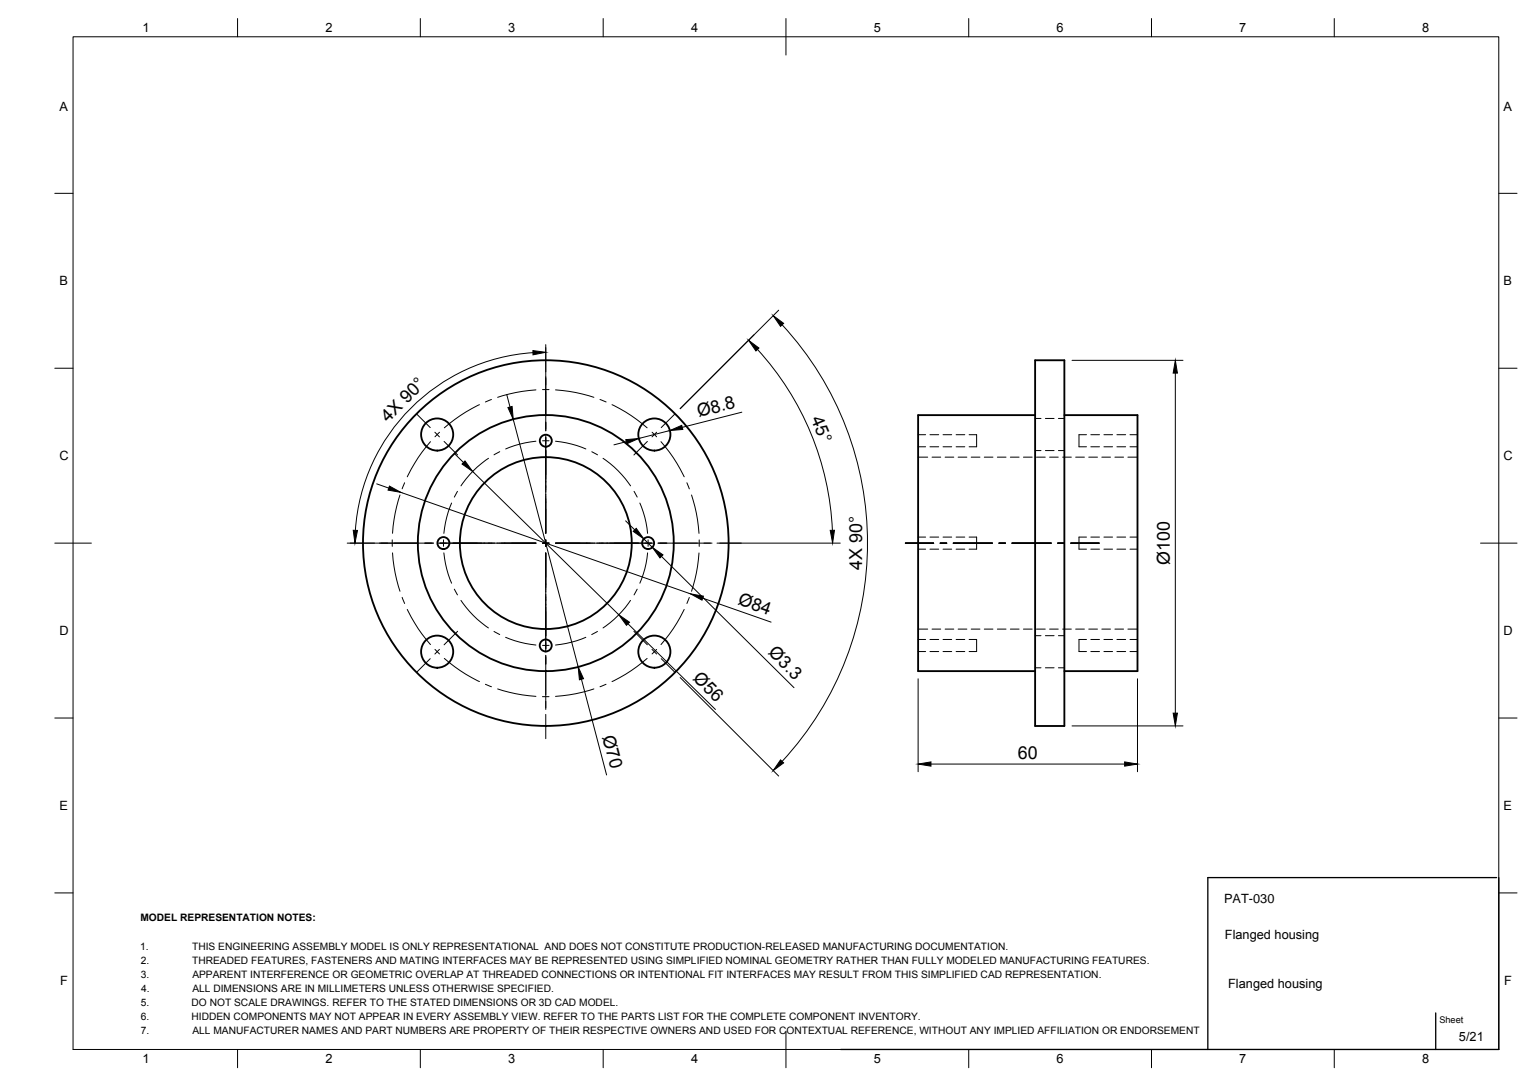
ISO-10303-21;
HEADER;
/* Generated by software containing ST-Developer
 * from STEP Tools, Inc. (www.steptools.com) 
 */

FILE_DESCRIPTION(
/* description */ ('Double-bearing flanged cartridge'),
/* implementation_level */ '2;1');

FILE_NAME(
/* name */ 'Flanged housing.step',
/* time_stamp */ '2026-10-28T03:26:40-07:00',
/* author */ (''),
/* organization */ (''),
/* preprocessor_version */ 'ST-DEVELOPER v20.2',
/* originating_system */ 'Autodesk Translation Framework v15.17.0.0',
/* authorisation */ '');

FILE_SCHEMA (('AUTOMOTIVE_DESIGN { 1 0 10303 214 3 1 1 }'));
ENDSEC;

DATA;
#10=MECHANICAL_DESIGN_GEOMETRIC_PRESENTATION_REPRESENTATION('',(#190),#5535);
#162=SHAPE_REPRESENTATION_RELATIONSHIP('SRR','None',#5603,#176);
#176=ADVANCED_BREP_SHAPE_REPRESENTATION('',(#212),#5519);
#190=STYLED_ITEM('',(#5743),#212);
#212=MANIFOLD_SOLID_BREP('Body1',#2324);
#233=FACE_BOUND('',#531,.T.);
#234=FACE_BOUND('',#532,.T.);
#235=FACE_BOUND('',#533,.T.);
#236=FACE_BOUND('',#534,.T.);
#237=FACE_BOUND('',#535,.T.);
#238=FACE_BOUND('',#537,.T.);
#239=FACE_BOUND('',#538,.T.);
#240=FACE_BOUND('',#539,.T.);
#241=FACE_BOUND('',#540,.T.);
#242=FACE_BOUND('',#541,.T.);
#243=FACE_BOUND('',#547,.T.);
#244=FACE_BOUND('',#548,.T.);
#245=FACE_BOUND('',#549,.T.);
#246=FACE_BOUND('',#550,.T.);
#247=FACE_BOUND('',#551,.T.);
#248=FACE_BOUND('',#553,.T.);
#249=FACE_BOUND('',#554,.T.);
#250=FACE_BOUND('',#555,.T.);
#251=FACE_BOUND('',#556,.T.);
#252=FACE_BOUND('',#557,.T.);
#300=PLANE('',#2520);
#301=PLANE('',#2524);
#302=PLANE('',#2528);
#303=PLANE('',#2532);
#304=PLANE('',#2536);
#305=PLANE('',#2540);
#306=PLANE('',#2544);
#307=PLANE('',#2548);
#308=PLANE('',#2549);
#309=PLANE('',#2552);
#310=PLANE('',#2563);
#311=PLANE('',#2564);
#361=FACE_OUTER_BOUND('',#510,.T.);
#362=FACE_OUTER_BOUND('',#511,.T.);
#363=FACE_OUTER_BOUND('',#512,.T.);
#364=FACE_OUTER_BOUND('',#513,.T.);
#365=FACE_OUTER_BOUND('',#514,.T.);
#366=FACE_OUTER_BOUND('',#515,.T.);
#367=FACE_OUTER_BOUND('',#516,.T.);
#368=FACE_OUTER_BOUND('',#517,.T.);
#369=FACE_OUTER_BOUND('',#518,.T.);
#370=FACE_OUTER_BOUND('',#519,.T.);
#371=FACE_OUTER_BOUND('',#520,.T.);
#372=FACE_OUTER_BOUND('',#521,.T.);
#373=FACE_OUTER_BOUND('',#522,.T.);
#374=FACE_OUTER_BOUND('',#523,.T.);
#375=FACE_OUTER_BOUND('',#524,.T.);
#376=FACE_OUTER_BOUND('',#525,.T.);
#377=FACE_OUTER_BOUND('',#526,.T.);
#378=FACE_OUTER_BOUND('',#527,.T.);
#379=FACE_OUTER_BOUND('',#528,.T.);
#380=FACE_OUTER_BOUND('',#529,.T.);
#381=FACE_OUTER_BOUND('',#530,.T.);
#382=FACE_OUTER_BOUND('',#536,.T.);
#383=FACE_OUTER_BOUND('',#542,.T.);
#384=FACE_OUTER_BOUND('',#543,.T.);
#385=FACE_OUTER_BOUND('',#544,.T.);
#386=FACE_OUTER_BOUND('',#545,.T.);
#387=FACE_OUTER_BOUND('',#546,.T.);
#388=FACE_OUTER_BOUND('',#552,.T.);
#510=EDGE_LOOP('',(#1550,#1551,#1552,#1553));
#511=EDGE_LOOP('',(#1554,#1555,#1556,#1557));
#512=EDGE_LOOP('',(#1558,#1559,#1560,#1561));
#513=EDGE_LOOP('',(#1562,#1563,#1564,#1565));
#514=EDGE_LOOP('',(#1566,#1567,#1568,#1569));
#515=EDGE_LOOP('',(#1570));
#516=EDGE_LOOP('',(#1571,#1572,#1573,#1574));
#517=EDGE_LOOP('',(#1575));
#518=EDGE_LOOP('',(#1576,#1577,#1578,#1579));
#519=EDGE_LOOP('',(#1580));
#520=EDGE_LOOP('',(#1581,#1582,#1583,#1584));
#521=EDGE_LOOP('',(#1585));
#522=EDGE_LOOP('',(#1586,#1587,#1588,#1589));
#523=EDGE_LOOP('',(#1590));
#524=EDGE_LOOP('',(#1591,#1592,#1593,#1594));
#525=EDGE_LOOP('',(#1595));
#526=EDGE_LOOP('',(#1596,#1597,#1598,#1599));
#527=EDGE_LOOP('',(#1600));
#528=EDGE_LOOP('',(#1601,#1602,#1603,#1604));
#529=EDGE_LOOP('',(#1605));
#530=EDGE_LOOP('',(#1606));
#531=EDGE_LOOP('',(#1607));
#532=EDGE_LOOP('',(#1608));
#533=EDGE_LOOP('',(#1609));
#534=EDGE_LOOP('',(#1610));
#535=EDGE_LOOP('',(#1611));
#536=EDGE_LOOP('',(#1612));
#537=EDGE_LOOP('',(#1613));
#538=EDGE_LOOP('',(#1614));
#539=EDGE_LOOP('',(#1615));
#540=EDGE_LOOP('',(#1616));
#541=EDGE_LOOP('',(#1617));
#542=EDGE_LOOP('',(#1618,#1619,#1620,#1621));
#543=EDGE_LOOP('',(#1622,#1623,#1624,#1625));
#544=EDGE_LOOP('',(#1626,#1627,#1628,#1629));
#545=EDGE_LOOP('',(#1630,#1631,#1632,#1633));
#546=EDGE_LOOP('',(#1634));
#547=EDGE_LOOP('',(#1635));
#548=EDGE_LOOP('',(#1636));
#549=EDGE_LOOP('',(#1637));
#550=EDGE_LOOP('',(#1638));
#551=EDGE_LOOP('',(#1639));
#552=EDGE_LOOP('',(#1640));
#553=EDGE_LOOP('',(#1641));
#554=EDGE_LOOP('',(#1642));
#555=EDGE_LOOP('',(#1643));
#556=EDGE_LOOP('',(#1644));
#557=EDGE_LOOP('',(#1645));
#726=LINE('',#3690,#812);
#727=LINE('',#3696,#813);
#728=LINE('',#3702,#814);
#729=LINE('',#3708,#815);
#730=LINE('',#3714,#816);
#731=LINE('',#3721,#817);
#732=LINE('',#3728,#818);
#733=LINE('',#3735,#819);
#734=LINE('',#3742,#820);
#735=LINE('',#3749,#821);
#736=LINE('',#3756,#822);
#737=LINE('',#3763,#823);
#738=LINE('',#3777,#824);
#739=LINE('',#3780,#825);
#740=LINE('',#3786,#826);
#741=LINE('',#3791,#827);
#812=VECTOR('',#2877,0.44);
#813=VECTOR('',#2884,0.44);
#814=VECTOR('',#2891,0.44);
#815=VECTOR('',#2898,0.44);
#816=VECTOR('',#2905,0.165);
#817=VECTOR('',#2914,0.165);
#818=VECTOR('',#2923,0.165);
#819=VECTOR('',#2932,0.165);
#820=VECTOR('',#2941,0.165);
#821=VECTOR('',#2950,0.165);
#822=VECTOR('',#2959,0.165);
#823=VECTOR('',#2968,0.165);
#824=VECTOR('',#2987,5.);
#825=VECTOR('',#2990,3.5);
#826=VECTOR('',#2997,2.35);
#827=VECTOR('',#3004,3.5);
#898=CIRCLE('',#2506,0.44);
#899=CIRCLE('',#2507,0.44);
#900=CIRCLE('',#2509,0.44);
#901=CIRCLE('',#2510,0.44);
#902=CIRCLE('',#2512,0.44);
#903=CIRCLE('',#2513,0.44);
#904=CIRCLE('',#2515,0.44);
#905=CIRCLE('',#2516,0.44);
#906=CIRCLE('',#2518,0.165);
#907=CIRCLE('',#2519,0.165);
#908=CIRCLE('',#2522,0.165);
#909=CIRCLE('',#2523,0.165);
#910=CIRCLE('',#2526,0.165);
#911=CIRCLE('',#2527,0.165);
#912=CIRCLE('',#2530,0.165);
#913=CIRCLE('',#2531,0.165);
#914=CIRCLE('',#2534,0.165);
#915=CIRCLE('',#2535,0.165);
#916=CIRCLE('',#2538,0.165);
#917=CIRCLE('',#2539,0.165);
#918=CIRCLE('',#2542,0.165);
#919=CIRCLE('',#2543,0.165);
#920=CIRCLE('',#2546,0.165);
#921=CIRCLE('',#2547,0.165);
#922=CIRCLE('',#2550,5.);
#923=CIRCLE('',#2551,3.5);
#924=CIRCLE('',#2553,5.);
#925=CIRCLE('',#2554,3.5);
#926=CIRCLE('',#2557,3.5);
#927=CIRCLE('',#2559,2.35);
#928=CIRCLE('',#2560,2.35);
#929=CIRCLE('',#2562,3.5);
#1072=VERTEX_POINT('',#3687);
#1073=VERTEX_POINT('',#3689);
#1074=VERTEX_POINT('',#3693);
#1075=VERTEX_POINT('',#3695);
#1076=VERTEX_POINT('',#3699);
#1077=VERTEX_POINT('',#3701);
#1078=VERTEX_POINT('',#3705);
#1079=VERTEX_POINT('',#3707);
#1080=VERTEX_POINT('',#3711);
#1081=VERTEX_POINT('',#3713);
#1082=VERTEX_POINT('',#3718);
#1083=VERTEX_POINT('',#3720);
#1084=VERTEX_POINT('',#3725);
#1085=VERTEX_POINT('',#3727);
#1086=VERTEX_POINT('',#3732);
#1087=VERTEX_POINT('',#3734);
#1088=VERTEX_POINT('',#3739);
#1089=VERTEX_POINT('',#3741);
#1090=VERTEX_POINT('',#3746);
#1091=VERTEX_POINT('',#3748);
#1092=VERTEX_POINT('',#3753);
#1093=VERTEX_POINT('',#3755);
#1094=VERTEX_POINT('',#3760);
#1095=VERTEX_POINT('',#3762);
#1096=VERTEX_POINT('',#3767);
#1097=VERTEX_POINT('',#3769);
#1098=VERTEX_POINT('',#3772);
#1099=VERTEX_POINT('',#3774);
#1100=VERTEX_POINT('',#3779);
#1101=VERTEX_POINT('',#3783);
#1102=VERTEX_POINT('',#3785);
#1103=VERTEX_POINT('',#3789);
#1268=EDGE_CURVE('',#1072,#1072,#898,.T.);
#1269=EDGE_CURVE('',#1072,#1073,#726,.T.);
#1270=EDGE_CURVE('',#1073,#1073,#899,.T.);
#1271=EDGE_CURVE('',#1074,#1074,#900,.T.);
#1272=EDGE_CURVE('',#1074,#1075,#727,.T.);
#1273=EDGE_CURVE('',#1075,#1075,#901,.T.);
#1274=EDGE_CURVE('',#1076,#1076,#902,.T.);
#1275=EDGE_CURVE('',#1076,#1077,#728,.T.);
#1276=EDGE_CURVE('',#1077,#1077,#903,.T.);
#1277=EDGE_CURVE('',#1078,#1078,#904,.T.);
#1278=EDGE_CURVE('',#1078,#1079,#729,.T.);
#1279=EDGE_CURVE('',#1079,#1079,#905,.T.);
#1280=EDGE_CURVE('',#1080,#1080,#906,.T.);
#1281=EDGE_CURVE('',#1080,#1081,#730,.T.);
#1282=EDGE_CURVE('',#1081,#1081,#907,.T.);
#1283=EDGE_CURVE('',#1082,#1082,#908,.T.);
#1284=EDGE_CURVE('',#1082,#1083,#731,.T.);
#1285=EDGE_CURVE('',#1083,#1083,#909,.T.);
#1286=EDGE_CURVE('',#1084,#1084,#910,.T.);
#1287=EDGE_CURVE('',#1084,#1085,#732,.T.);
#1288=EDGE_CURVE('',#1085,#1085,#911,.T.);
#1289=EDGE_CURVE('',#1086,#1086,#912,.T.);
#1290=EDGE_CURVE('',#1086,#1087,#733,.T.);
#1291=EDGE_CURVE('',#1087,#1087,#913,.T.);
#1292=EDGE_CURVE('',#1088,#1088,#914,.T.);
#1293=EDGE_CURVE('',#1088,#1089,#734,.T.);
#1294=EDGE_CURVE('',#1089,#1089,#915,.T.);
#1295=EDGE_CURVE('',#1090,#1090,#916,.T.);
#1296=EDGE_CURVE('',#1090,#1091,#735,.T.);
#1297=EDGE_CURVE('',#1091,#1091,#917,.T.);
#1298=EDGE_CURVE('',#1092,#1092,#918,.T.);
#1299=EDGE_CURVE('',#1092,#1093,#736,.T.);
#1300=EDGE_CURVE('',#1093,#1093,#919,.T.);
#1301=EDGE_CURVE('',#1094,#1094,#920,.T.);
#1302=EDGE_CURVE('',#1094,#1095,#737,.T.);
#1303=EDGE_CURVE('',#1095,#1095,#921,.T.);
#1304=EDGE_CURVE('',#1096,#1096,#922,.T.);
#1305=EDGE_CURVE('',#1097,#1097,#923,.T.);
#1306=EDGE_CURVE('',#1098,#1098,#924,.T.);
#1307=EDGE_CURVE('',#1099,#1099,#925,.T.);
#1308=EDGE_CURVE('',#1096,#1098,#738,.T.);
#1309=EDGE_CURVE('',#1099,#1100,#739,.T.);
#1310=EDGE_CURVE('',#1100,#1100,#926,.T.);
#1311=EDGE_CURVE('',#1101,#1101,#927,.T.);
#1312=EDGE_CURVE('',#1101,#1102,#740,.T.);
#1313=EDGE_CURVE('',#1102,#1102,#928,.T.);
#1314=EDGE_CURVE('',#1103,#1103,#929,.T.);
#1315=EDGE_CURVE('',#1103,#1097,#741,.T.);
#1550=ORIENTED_EDGE('',*,*,#1268,.F.);
#1551=ORIENTED_EDGE('',*,*,#1269,.T.);
#1552=ORIENTED_EDGE('',*,*,#1270,.F.);
#1553=ORIENTED_EDGE('',*,*,#1269,.F.);
#1554=ORIENTED_EDGE('',*,*,#1271,.F.);
#1555=ORIENTED_EDGE('',*,*,#1272,.T.);
#1556=ORIENTED_EDGE('',*,*,#1273,.F.);
#1557=ORIENTED_EDGE('',*,*,#1272,.F.);
#1558=ORIENTED_EDGE('',*,*,#1274,.F.);
#1559=ORIENTED_EDGE('',*,*,#1275,.T.);
#1560=ORIENTED_EDGE('',*,*,#1276,.F.);
#1561=ORIENTED_EDGE('',*,*,#1275,.F.);
#1562=ORIENTED_EDGE('',*,*,#1277,.F.);
#1563=ORIENTED_EDGE('',*,*,#1278,.T.);
#1564=ORIENTED_EDGE('',*,*,#1279,.F.);
#1565=ORIENTED_EDGE('',*,*,#1278,.F.);
#1566=ORIENTED_EDGE('',*,*,#1280,.F.);
#1567=ORIENTED_EDGE('',*,*,#1281,.T.);
#1568=ORIENTED_EDGE('',*,*,#1282,.F.);
#1569=ORIENTED_EDGE('',*,*,#1281,.F.);
#1570=ORIENTED_EDGE('',*,*,#1280,.T.);
#1571=ORIENTED_EDGE('',*,*,#1283,.F.);
#1572=ORIENTED_EDGE('',*,*,#1284,.T.);
#1573=ORIENTED_EDGE('',*,*,#1285,.F.);
#1574=ORIENTED_EDGE('',*,*,#1284,.F.);
#1575=ORIENTED_EDGE('',*,*,#1283,.T.);
#1576=ORIENTED_EDGE('',*,*,#1286,.F.);
#1577=ORIENTED_EDGE('',*,*,#1287,.T.);
#1578=ORIENTED_EDGE('',*,*,#1288,.F.);
#1579=ORIENTED_EDGE('',*,*,#1287,.F.);
#1580=ORIENTED_EDGE('',*,*,#1286,.T.);
#1581=ORIENTED_EDGE('',*,*,#1289,.F.);
#1582=ORIENTED_EDGE('',*,*,#1290,.T.);
#1583=ORIENTED_EDGE('',*,*,#1291,.F.);
#1584=ORIENTED_EDGE('',*,*,#1290,.F.);
#1585=ORIENTED_EDGE('',*,*,#1289,.T.);
#1586=ORIENTED_EDGE('',*,*,#1292,.F.);
#1587=ORIENTED_EDGE('',*,*,#1293,.T.);
#1588=ORIENTED_EDGE('',*,*,#1294,.T.);
#1589=ORIENTED_EDGE('',*,*,#1293,.F.);
#1590=ORIENTED_EDGE('',*,*,#1294,.F.);
#1591=ORIENTED_EDGE('',*,*,#1295,.F.);
#1592=ORIENTED_EDGE('',*,*,#1296,.T.);
#1593=ORIENTED_EDGE('',*,*,#1297,.T.);
#1594=ORIENTED_EDGE('',*,*,#1296,.F.);
#1595=ORIENTED_EDGE('',*,*,#1297,.F.);
#1596=ORIENTED_EDGE('',*,*,#1298,.F.);
#1597=ORIENTED_EDGE('',*,*,#1299,.T.);
#1598=ORIENTED_EDGE('',*,*,#1300,.T.);
#1599=ORIENTED_EDGE('',*,*,#1299,.F.);
#1600=ORIENTED_EDGE('',*,*,#1300,.F.);
#1601=ORIENTED_EDGE('',*,*,#1301,.F.);
#1602=ORIENTED_EDGE('',*,*,#1302,.T.);
#1603=ORIENTED_EDGE('',*,*,#1303,.T.);
#1604=ORIENTED_EDGE('',*,*,#1302,.F.);
#1605=ORIENTED_EDGE('',*,*,#1303,.F.);
#1606=ORIENTED_EDGE('',*,*,#1304,.T.);
#1607=ORIENTED_EDGE('',*,*,#1305,.F.);
#1608=ORIENTED_EDGE('',*,*,#1279,.T.);
#1609=ORIENTED_EDGE('',*,*,#1276,.T.);
#1610=ORIENTED_EDGE('',*,*,#1273,.T.);
#1611=ORIENTED_EDGE('',*,*,#1270,.T.);
#1612=ORIENTED_EDGE('',*,*,#1306,.F.);
#1613=ORIENTED_EDGE('',*,*,#1307,.F.);
#1614=ORIENTED_EDGE('',*,*,#1277,.T.);
#1615=ORIENTED_EDGE('',*,*,#1274,.T.);
#1616=ORIENTED_EDGE('',*,*,#1271,.T.);
#1617=ORIENTED_EDGE('',*,*,#1268,.T.);
#1618=ORIENTED_EDGE('',*,*,#1304,.F.);
#1619=ORIENTED_EDGE('',*,*,#1308,.T.);
#1620=ORIENTED_EDGE('',*,*,#1306,.T.);
#1621=ORIENTED_EDGE('',*,*,#1308,.F.);
#1622=ORIENTED_EDGE('',*,*,#1307,.T.);
#1623=ORIENTED_EDGE('',*,*,#1309,.T.);
#1624=ORIENTED_EDGE('',*,*,#1310,.T.);
#1625=ORIENTED_EDGE('',*,*,#1309,.F.);
#1626=ORIENTED_EDGE('',*,*,#1311,.F.);
#1627=ORIENTED_EDGE('',*,*,#1312,.T.);
#1628=ORIENTED_EDGE('',*,*,#1313,.T.);
#1629=ORIENTED_EDGE('',*,*,#1312,.F.);
#1630=ORIENTED_EDGE('',*,*,#1314,.F.);
#1631=ORIENTED_EDGE('',*,*,#1315,.T.);
#1632=ORIENTED_EDGE('',*,*,#1305,.T.);
#1633=ORIENTED_EDGE('',*,*,#1315,.F.);
#1634=ORIENTED_EDGE('',*,*,#1314,.T.);
#1635=ORIENTED_EDGE('',*,*,#1311,.T.);
#1636=ORIENTED_EDGE('',*,*,#1291,.T.);
#1637=ORIENTED_EDGE('',*,*,#1288,.T.);
#1638=ORIENTED_EDGE('',*,*,#1285,.T.);
#1639=ORIENTED_EDGE('',*,*,#1282,.T.);
#1640=ORIENTED_EDGE('',*,*,#1310,.F.);
#1641=ORIENTED_EDGE('',*,*,#1313,.F.);
#1642=ORIENTED_EDGE('',*,*,#1301,.T.);
#1643=ORIENTED_EDGE('',*,*,#1298,.T.);
#1644=ORIENTED_EDGE('',*,*,#1295,.T.);
#1645=ORIENTED_EDGE('',*,*,#1292,.T.);
#2114=CYLINDRICAL_SURFACE('',#2505,0.44);
#2115=CYLINDRICAL_SURFACE('',#2508,0.44);
#2116=CYLINDRICAL_SURFACE('',#2511,0.44);
#2117=CYLINDRICAL_SURFACE('',#2514,0.44);
#2118=CYLINDRICAL_SURFACE('',#2517,0.165);
#2119=CYLINDRICAL_SURFACE('',#2521,0.165);
#2120=CYLINDRICAL_SURFACE('',#2525,0.165);
#2121=CYLINDRICAL_SURFACE('',#2529,0.165);
#2122=CYLINDRICAL_SURFACE('',#2533,0.165);
#2123=CYLINDRICAL_SURFACE('',#2537,0.165);
#2124=CYLINDRICAL_SURFACE('',#2541,0.165);
#2125=CYLINDRICAL_SURFACE('',#2545,0.165);
#2126=CYLINDRICAL_SURFACE('',#2555,5.);
#2127=CYLINDRICAL_SURFACE('',#2556,3.5);
#2128=CYLINDRICAL_SURFACE('',#2558,2.35);
#2129=CYLINDRICAL_SURFACE('',#2561,3.5);
#2175=ADVANCED_FACE('',(#361),#2114,.F.);
#2176=ADVANCED_FACE('',(#362),#2115,.F.);
#2177=ADVANCED_FACE('',(#363),#2116,.F.);
#2178=ADVANCED_FACE('',(#364),#2117,.F.);
#2179=ADVANCED_FACE('',(#365),#2118,.F.);
#2180=ADVANCED_FACE('',(#366),#300,.T.);
#2181=ADVANCED_FACE('',(#367),#2119,.F.);
#2182=ADVANCED_FACE('',(#368),#301,.T.);
#2183=ADVANCED_FACE('',(#369),#2120,.F.);
#2184=ADVANCED_FACE('',(#370),#302,.T.);
#2185=ADVANCED_FACE('',(#371),#2121,.F.);
#2186=ADVANCED_FACE('',(#372),#303,.T.);
#2187=ADVANCED_FACE('',(#373),#2122,.F.);
#2188=ADVANCED_FACE('',(#374),#304,.F.);
#2189=ADVANCED_FACE('',(#375),#2123,.F.);
#2190=ADVANCED_FACE('',(#376),#305,.F.);
#2191=ADVANCED_FACE('',(#377),#2124,.F.);
#2192=ADVANCED_FACE('',(#378),#306,.F.);
#2193=ADVANCED_FACE('',(#379),#2125,.F.);
#2194=ADVANCED_FACE('',(#380),#307,.F.);
#2195=ADVANCED_FACE('',(#381,#233,#234,#235,#236,#237),#308,.T.);
#2196=ADVANCED_FACE('',(#382,#238,#239,#240,#241,#242),#309,.F.);
#2197=ADVANCED_FACE('',(#383),#2126,.T.);
#2198=ADVANCED_FACE('',(#384),#2127,.T.);
#2199=ADVANCED_FACE('',(#385),#2128,.F.);
#2200=ADVANCED_FACE('',(#386),#2129,.T.);
#2201=ADVANCED_FACE('',(#387,#243,#244,#245,#246,#247),#310,.T.);
#2202=ADVANCED_FACE('',(#388,#248,#249,#250,#251,#252),#311,.F.);
#2324=CLOSED_SHELL('',(#2175,#2176,#2177,#2178,#2179,#2180,#2181,#2182,
#2183,#2184,#2185,#2186,#2187,#2188,#2189,#2190,#2191,#2192,#2193,#2194,
#2195,#2196,#2197,#2198,#2199,#2200,#2201,#2202));
#2504=AXIS2_PLACEMENT_3D('',#3685,#2871,#2872);
#2505=AXIS2_PLACEMENT_3D('',#3686,#2873,#2874);
#2506=AXIS2_PLACEMENT_3D('',#3688,#2875,#2876);
#2507=AXIS2_PLACEMENT_3D('',#3691,#2878,#2879);
#2508=AXIS2_PLACEMENT_3D('',#3692,#2880,#2881);
#2509=AXIS2_PLACEMENT_3D('',#3694,#2882,#2883);
#2510=AXIS2_PLACEMENT_3D('',#3697,#2885,#2886);
#2511=AXIS2_PLACEMENT_3D('',#3698,#2887,#2888);
#2512=AXIS2_PLACEMENT_3D('',#3700,#2889,#2890);
#2513=AXIS2_PLACEMENT_3D('',#3703,#2892,#2893);
#2514=AXIS2_PLACEMENT_3D('',#3704,#2894,#2895);
#2515=AXIS2_PLACEMENT_3D('',#3706,#2896,#2897);
#2516=AXIS2_PLACEMENT_3D('',#3709,#2899,#2900);
#2517=AXIS2_PLACEMENT_3D('',#3710,#2901,#2902);
#2518=AXIS2_PLACEMENT_3D('',#3712,#2903,#2904);
#2519=AXIS2_PLACEMENT_3D('',#3715,#2906,#2907);
#2520=AXIS2_PLACEMENT_3D('',#3716,#2908,#2909);
#2521=AXIS2_PLACEMENT_3D('',#3717,#2910,#2911);
#2522=AXIS2_PLACEMENT_3D('',#3719,#2912,#2913);
#2523=AXIS2_PLACEMENT_3D('',#3722,#2915,#2916);
#2524=AXIS2_PLACEMENT_3D('',#3723,#2917,#2918);
#2525=AXIS2_PLACEMENT_3D('',#3724,#2919,#2920);
#2526=AXIS2_PLACEMENT_3D('',#3726,#2921,#2922);
#2527=AXIS2_PLACEMENT_3D('',#3729,#2924,#2925);
#2528=AXIS2_PLACEMENT_3D('',#3730,#2926,#2927);
#2529=AXIS2_PLACEMENT_3D('',#3731,#2928,#2929);
#2530=AXIS2_PLACEMENT_3D('',#3733,#2930,#2931);
#2531=AXIS2_PLACEMENT_3D('',#3736,#2933,#2934);
#2532=AXIS2_PLACEMENT_3D('',#3737,#2935,#2936);
#2533=AXIS2_PLACEMENT_3D('',#3738,#2937,#2938);
#2534=AXIS2_PLACEMENT_3D('',#3740,#2939,#2940);
#2535=AXIS2_PLACEMENT_3D('',#3743,#2942,#2943);
#2536=AXIS2_PLACEMENT_3D('',#3744,#2944,#2945);
#2537=AXIS2_PLACEMENT_3D('',#3745,#2946,#2947);
#2538=AXIS2_PLACEMENT_3D('',#3747,#2948,#2949);
#2539=AXIS2_PLACEMENT_3D('',#3750,#2951,#2952);
#2540=AXIS2_PLACEMENT_3D('',#3751,#2953,#2954);
#2541=AXIS2_PLACEMENT_3D('',#3752,#2955,#2956);
#2542=AXIS2_PLACEMENT_3D('',#3754,#2957,#2958);
#2543=AXIS2_PLACEMENT_3D('',#3757,#2960,#2961);
#2544=AXIS2_PLACEMENT_3D('',#3758,#2962,#2963);
#2545=AXIS2_PLACEMENT_3D('',#3759,#2964,#2965);
#2546=AXIS2_PLACEMENT_3D('',#3761,#2966,#2967);
#2547=AXIS2_PLACEMENT_3D('',#3764,#2969,#2970);
#2548=AXIS2_PLACEMENT_3D('',#3765,#2971,#2972);
#2549=AXIS2_PLACEMENT_3D('',#3766,#2973,#2974);
#2550=AXIS2_PLACEMENT_3D('',#3768,#2975,#2976);
#2551=AXIS2_PLACEMENT_3D('',#3770,#2977,#2978);
#2552=AXIS2_PLACEMENT_3D('',#3771,#2979,#2980);
#2553=AXIS2_PLACEMENT_3D('',#3773,#2981,#2982);
#2554=AXIS2_PLACEMENT_3D('',#3775,#2983,#2984);
#2555=AXIS2_PLACEMENT_3D('',#3776,#2985,#2986);
#2556=AXIS2_PLACEMENT_3D('',#3778,#2988,#2989);
#2557=AXIS2_PLACEMENT_3D('',#3781,#2991,#2992);
#2558=AXIS2_PLACEMENT_3D('',#3782,#2993,#2994);
#2559=AXIS2_PLACEMENT_3D('',#3784,#2995,#2996);
#2560=AXIS2_PLACEMENT_3D('',#3787,#2998,#2999);
#2561=AXIS2_PLACEMENT_3D('',#3788,#3000,#3001);
#2562=AXIS2_PLACEMENT_3D('',#3790,#3002,#3003);
#2563=AXIS2_PLACEMENT_3D('',#3792,#3005,#3006);
#2564=AXIS2_PLACEMENT_3D('',#3793,#3007,#3008);
#2871=DIRECTION('axis',(0.,0.,1.));
#2872=DIRECTION('refdir',(1.,0.,0.));
#2873=DIRECTION('center_axis',(0.,1.,0.));
#2874=DIRECTION('ref_axis',(1.,0.,0.));
#2875=DIRECTION('center_axis',(0.,1.,0.));
#2876=DIRECTION('ref_axis',(1.,0.,0.));
#2877=DIRECTION('',(0.,1.,0.));
#2878=DIRECTION('center_axis',(0.,-1.,0.));
#2879=DIRECTION('ref_axis',(1.,0.,0.));
#2880=DIRECTION('center_axis',(0.,1.,0.));
#2881=DIRECTION('ref_axis',(1.,0.,0.));
#2882=DIRECTION('center_axis',(0.,1.,0.));
#2883=DIRECTION('ref_axis',(1.,0.,0.));
#2884=DIRECTION('',(0.,1.,0.));
#2885=DIRECTION('center_axis',(0.,-1.,0.));
#2886=DIRECTION('ref_axis',(1.,0.,0.));
#2887=DIRECTION('center_axis',(0.,1.,0.));
#2888=DIRECTION('ref_axis',(1.,0.,0.));
#2889=DIRECTION('center_axis',(0.,1.,0.));
#2890=DIRECTION('ref_axis',(1.,0.,0.));
#2891=DIRECTION('',(0.,1.,0.));
#2892=DIRECTION('center_axis',(0.,-1.,0.));
#2893=DIRECTION('ref_axis',(1.,0.,0.));
#2894=DIRECTION('center_axis',(0.,1.,0.));
#2895=DIRECTION('ref_axis',(1.,0.,0.));
#2896=DIRECTION('center_axis',(0.,1.,0.));
#2897=DIRECTION('ref_axis',(1.,0.,0.));
#2898=DIRECTION('',(0.,1.,0.));
#2899=DIRECTION('center_axis',(0.,-1.,0.));
#2900=DIRECTION('ref_axis',(1.,0.,0.));
#2901=DIRECTION('center_axis',(0.,1.,0.));
#2902=DIRECTION('ref_axis',(1.,0.,0.));
#2903=DIRECTION('center_axis',(0.,1.,0.));
#2904=DIRECTION('ref_axis',(1.,0.,0.));
#2905=DIRECTION('',(0.,1.,0.));
#2906=DIRECTION('center_axis',(0.,-1.,0.));
#2907=DIRECTION('ref_axis',(1.,0.,0.));
#2908=DIRECTION('center_axis',(0.,1.,0.));
#2909=DIRECTION('ref_axis',(1.,0.,0.));
#2910=DIRECTION('center_axis',(0.,1.,0.));
#2911=DIRECTION('ref_axis',(1.,0.,0.));
#2912=DIRECTION('center_axis',(0.,1.,0.));
#2913=DIRECTION('ref_axis',(1.,0.,0.));
#2914=DIRECTION('',(0.,1.,0.));
#2915=DIRECTION('center_axis',(0.,-1.,0.));
#2916=DIRECTION('ref_axis',(1.,0.,0.));
#2917=DIRECTION('center_axis',(0.,1.,0.));
#2918=DIRECTION('ref_axis',(1.,0.,0.));
#2919=DIRECTION('center_axis',(0.,1.,0.));
#2920=DIRECTION('ref_axis',(1.,0.,0.));
#2921=DIRECTION('center_axis',(0.,1.,0.));
#2922=DIRECTION('ref_axis',(1.,0.,0.));
#2923=DIRECTION('',(0.,1.,0.));
#2924=DIRECTION('center_axis',(0.,-1.,0.));
#2925=DIRECTION('ref_axis',(1.,0.,0.));
#2926=DIRECTION('center_axis',(0.,1.,0.));
#2927=DIRECTION('ref_axis',(1.,0.,0.));
#2928=DIRECTION('center_axis',(0.,1.,0.));
#2929=DIRECTION('ref_axis',(1.,0.,0.));
#2930=DIRECTION('center_axis',(0.,1.,0.));
#2931=DIRECTION('ref_axis',(1.,0.,0.));
#2932=DIRECTION('',(0.,1.,0.));
#2933=DIRECTION('center_axis',(0.,-1.,0.));
#2934=DIRECTION('ref_axis',(1.,0.,0.));
#2935=DIRECTION('center_axis',(0.,1.,0.));
#2936=DIRECTION('ref_axis',(1.,0.,0.));
#2937=DIRECTION('center_axis',(0.,1.,0.));
#2938=DIRECTION('ref_axis',(1.,0.,0.));
#2939=DIRECTION('center_axis',(0.,1.,0.));
#2940=DIRECTION('ref_axis',(1.,0.,0.));
#2941=DIRECTION('',(0.,1.,0.));
#2942=DIRECTION('center_axis',(0.,1.,0.));
#2943=DIRECTION('ref_axis',(1.,0.,0.));
#2944=DIRECTION('center_axis',(0.,1.,0.));
#2945=DIRECTION('ref_axis',(1.,0.,0.));
#2946=DIRECTION('center_axis',(0.,1.,0.));
#2947=DIRECTION('ref_axis',(1.,0.,0.));
#2948=DIRECTION('center_axis',(0.,1.,0.));
#2949=DIRECTION('ref_axis',(1.,0.,0.));
#2950=DIRECTION('',(0.,1.,0.));
#2951=DIRECTION('center_axis',(0.,1.,0.));
#2952=DIRECTION('ref_axis',(1.,0.,0.));
#2953=DIRECTION('center_axis',(0.,1.,0.));
#2954=DIRECTION('ref_axis',(1.,0.,0.));
#2955=DIRECTION('center_axis',(0.,1.,0.));
#2956=DIRECTION('ref_axis',(1.,0.,0.));
#2957=DIRECTION('center_axis',(0.,1.,0.));
#2958=DIRECTION('ref_axis',(1.,0.,0.));
#2959=DIRECTION('',(0.,1.,0.));
#2960=DIRECTION('center_axis',(0.,1.,0.));
#2961=DIRECTION('ref_axis',(1.,0.,0.));
#2962=DIRECTION('center_axis',(0.,1.,0.));
#2963=DIRECTION('ref_axis',(1.,0.,0.));
#2964=DIRECTION('center_axis',(0.,1.,0.));
#2965=DIRECTION('ref_axis',(1.,0.,0.));
#2966=DIRECTION('center_axis',(0.,1.,0.));
#2967=DIRECTION('ref_axis',(1.,0.,0.));
#2968=DIRECTION('',(0.,1.,0.));
#2969=DIRECTION('center_axis',(0.,1.,0.));
#2970=DIRECTION('ref_axis',(1.,0.,0.));
#2971=DIRECTION('center_axis',(0.,1.,0.));
#2972=DIRECTION('ref_axis',(1.,0.,0.));
#2973=DIRECTION('center_axis',(0.,1.,0.));
#2974=DIRECTION('ref_axis',(1.,0.,0.));
#2975=DIRECTION('center_axis',(0.,1.,0.));
#2976=DIRECTION('ref_axis',(1.,0.,0.));
#2977=DIRECTION('center_axis',(0.,1.,0.));
#2978=DIRECTION('ref_axis',(1.,0.,0.));
#2979=DIRECTION('center_axis',(0.,1.,0.));
#2980=DIRECTION('ref_axis',(1.,0.,0.));
#2981=DIRECTION('center_axis',(0.,1.,0.));
#2982=DIRECTION('ref_axis',(1.,0.,0.));
#2983=DIRECTION('center_axis',(0.,-1.,0.));
#2984=DIRECTION('ref_axis',(1.,0.,0.));
#2985=DIRECTION('center_axis',(0.,1.,0.));
#2986=DIRECTION('ref_axis',(1.,0.,0.));
#2987=DIRECTION('',(0.,-1.,0.));
#2988=DIRECTION('center_axis',(0.,1.,0.));
#2989=DIRECTION('ref_axis',(1.,0.,0.));
#2990=DIRECTION('',(0.,-1.,0.));
#2991=DIRECTION('center_axis',(0.,1.,0.));
#2992=DIRECTION('ref_axis',(1.,0.,0.));
#2993=DIRECTION('center_axis',(0.,1.,0.));
#2994=DIRECTION('ref_axis',(1.,0.,0.));
#2995=DIRECTION('center_axis',(0.,-1.,0.));
#2996=DIRECTION('ref_axis',(1.,0.,0.));
#2997=DIRECTION('',(0.,-1.,0.));
#2998=DIRECTION('center_axis',(0.,-1.,0.));
#2999=DIRECTION('ref_axis',(1.,0.,0.));
#3000=DIRECTION('center_axis',(0.,1.,0.));
#3001=DIRECTION('ref_axis',(1.,0.,0.));
#3002=DIRECTION('center_axis',(0.,1.,0.));
#3003=DIRECTION('ref_axis',(1.,0.,0.));
#3004=DIRECTION('',(0.,-1.,0.));
#3005=DIRECTION('center_axis',(0.,1.,0.));
#3006=DIRECTION('ref_axis',(1.,0.,0.));
#3007=DIRECTION('center_axis',(0.,1.,0.));
#3008=DIRECTION('ref_axis',(1.,0.,0.));
#3685=CARTESIAN_POINT('',(0.,0.,0.));
#3686=CARTESIAN_POINT('Origin',(-2.9698484809835,1.9,1.5301515190165));
#3687=CARTESIAN_POINT('',(-3.4098484809835,2.,1.5301515190165));
#3688=CARTESIAN_POINT('Origin',(-2.9698484809835,2.,1.5301515190165));
#3689=CARTESIAN_POINT('',(-3.4098484809835,2.8,1.5301515190165));
#3690=CARTESIAN_POINT('',(-3.4098484809835,1.9,1.5301515190165));
#3691=CARTESIAN_POINT('Origin',(-2.9698484809835,2.8,1.5301515190165));
#3692=CARTESIAN_POINT('Origin',(-2.9698484809835,1.9,7.4698484809835));
#3693=CARTESIAN_POINT('',(-3.4098484809835,2.,7.4698484809835));
#3694=CARTESIAN_POINT('Origin',(-2.9698484809835,2.,7.4698484809835));
#3695=CARTESIAN_POINT('',(-3.4098484809835,2.8,7.4698484809835));
#3696=CARTESIAN_POINT('',(-3.4098484809835,1.9,7.4698484809835));
#3697=CARTESIAN_POINT('Origin',(-2.9698484809835,2.8,7.4698484809835));
#3698=CARTESIAN_POINT('Origin',(2.9698484809835,1.9,7.4698484809835));
#3699=CARTESIAN_POINT('',(2.5298484809835,2.,7.4698484809835));
#3700=CARTESIAN_POINT('Origin',(2.9698484809835,2.,7.4698484809835));
#3701=CARTESIAN_POINT('',(2.5298484809835,2.8,7.4698484809835));
#3702=CARTESIAN_POINT('',(2.5298484809835,1.9,7.4698484809835));
#3703=CARTESIAN_POINT('Origin',(2.9698484809835,2.8,7.4698484809835));
#3704=CARTESIAN_POINT('Origin',(2.9698484809835,1.9,1.5301515190165));
#3705=CARTESIAN_POINT('',(2.5298484809835,2.,1.5301515190165));
#3706=CARTESIAN_POINT('Origin',(2.9698484809835,2.,1.5301515190165));
#3707=CARTESIAN_POINT('',(2.5298484809835,2.8,1.5301515190165));
#3708=CARTESIAN_POINT('',(2.5298484809835,1.9,1.5301515190165));
#3709=CARTESIAN_POINT('Origin',(2.9698484809835,2.8,1.5301515190165));
#3710=CARTESIAN_POINT('Origin',(-2.8,4.4,4.5));
#3711=CARTESIAN_POINT('',(-2.965,4.4,4.5));
#3712=CARTESIAN_POINT('Origin',(-2.8,4.4,4.5));
#3713=CARTESIAN_POINT('',(-2.965,6.,4.5));
#3714=CARTESIAN_POINT('',(-2.965,4.4,4.5));
#3715=CARTESIAN_POINT('Origin',(-2.8,6.,4.5));
#3716=CARTESIAN_POINT('Origin',(-2.8,4.4,4.5));
#3717=CARTESIAN_POINT('Origin',(1.71450551880629E-16,4.4,7.3));
#3718=CARTESIAN_POINT('',(-0.165,4.4,7.3));
#3719=CARTESIAN_POINT('Origin',(1.71450551880629E-16,4.4,7.3));
#3720=CARTESIAN_POINT('',(-0.165,6.,7.3));
#3721=CARTESIAN_POINT('',(-0.165,4.4,7.3));
#3722=CARTESIAN_POINT('Origin',(1.71450551880629E-16,6.,7.3));
#3723=CARTESIAN_POINT('Origin',(1.66533453693773E-16,4.4,7.3));
#3724=CARTESIAN_POINT('Origin',(2.8,4.4,4.5));
#3725=CARTESIAN_POINT('',(2.635,4.4,4.5));
#3726=CARTESIAN_POINT('Origin',(2.8,4.4,4.5));
#3727=CARTESIAN_POINT('',(2.635,6.,4.5));
#3728=CARTESIAN_POINT('',(2.635,4.4,4.5));
#3729=CARTESIAN_POINT('Origin',(2.8,6.,4.5));
#3730=CARTESIAN_POINT('Origin',(2.8,4.4,4.5));
#3731=CARTESIAN_POINT('Origin',(-5.14351655641888E-16,4.4,1.7));
#3732=CARTESIAN_POINT('',(-0.165000000000001,4.4,1.7));
#3733=CARTESIAN_POINT('Origin',(-5.14351655641888E-16,4.4,1.7));
#3734=CARTESIAN_POINT('',(-0.165000000000001,6.,1.7));
#3735=CARTESIAN_POINT('',(-0.165000000000001,4.4,1.7));
#3736=CARTESIAN_POINT('Origin',(-5.14351655641888E-16,6.,1.7));
#3737=CARTESIAN_POINT('Origin',(-5.27355936696949E-16,4.4,1.7));
#3738=CARTESIAN_POINT('Origin',(-2.8,-0.1,4.5));
#3739=CARTESIAN_POINT('',(-2.965,0.,4.5));
#3740=CARTESIAN_POINT('Origin',(-2.8,0.,4.5));
#3741=CARTESIAN_POINT('',(-2.965,1.6,4.5));
#3742=CARTESIAN_POINT('',(-2.965,-0.1,4.5));
#3743=CARTESIAN_POINT('Origin',(-2.8,1.6,4.5));
#3744=CARTESIAN_POINT('Origin',(-2.8,1.6,4.5));
#3745=CARTESIAN_POINT('Origin',(1.71450551880629E-16,-0.1,7.3));
#3746=CARTESIAN_POINT('',(-0.165,0.,7.3));
#3747=CARTESIAN_POINT('Origin',(1.71450551880629E-16,0.,7.3));
#3748=CARTESIAN_POINT('',(-0.165,1.6,7.3));
#3749=CARTESIAN_POINT('',(-0.165,-0.1,7.3));
#3750=CARTESIAN_POINT('Origin',(1.71450551880629E-16,1.6,7.3));
#3751=CARTESIAN_POINT('Origin',(1.66533453693773E-16,1.6,7.3));
#3752=CARTESIAN_POINT('Origin',(2.8,-0.1,4.5));
#3753=CARTESIAN_POINT('',(2.635,0.,4.5));
#3754=CARTESIAN_POINT('Origin',(2.8,0.,4.5));
#3755=CARTESIAN_POINT('',(2.635,1.6,4.5));
#3756=CARTESIAN_POINT('',(2.635,-0.1,4.5));
#3757=CARTESIAN_POINT('Origin',(2.8,1.6,4.5));
#3758=CARTESIAN_POINT('Origin',(2.8,1.6,4.5));
#3759=CARTESIAN_POINT('Origin',(-5.14351655641888E-16,-0.1,1.7));
#3760=CARTESIAN_POINT('',(-0.165000000000001,0.,1.7));
#3761=CARTESIAN_POINT('Origin',(-5.14351655641888E-16,0.,1.7));
#3762=CARTESIAN_POINT('',(-0.165000000000001,1.6,1.7));
#3763=CARTESIAN_POINT('',(-0.165000000000001,-0.1,1.7));
#3764=CARTESIAN_POINT('Origin',(-5.14351655641888E-16,1.6,1.7));
#3765=CARTESIAN_POINT('Origin',(-5.27355936696949E-16,1.6,1.7));
#3766=CARTESIAN_POINT('Origin',(0.,2.8,4.5));
#3767=CARTESIAN_POINT('',(-5.,2.8,4.5));
#3768=CARTESIAN_POINT('Origin',(0.,2.8,4.5));
#3769=CARTESIAN_POINT('',(-3.5,2.8,4.5));
#3770=CARTESIAN_POINT('Origin',(0.,2.8,4.5));
#3771=CARTESIAN_POINT('Origin',(0.,2.,4.5));
#3772=CARTESIAN_POINT('',(-5.,2.,4.5));
#3773=CARTESIAN_POINT('Origin',(0.,2.,4.5));
#3774=CARTESIAN_POINT('',(-3.5,2.,4.5));
#3775=CARTESIAN_POINT('Origin',(0.,2.,4.5));
#3776=CARTESIAN_POINT('Origin',(0.,2.,4.5));
#3777=CARTESIAN_POINT('',(-5.,2.,4.5));
#3778=CARTESIAN_POINT('Origin',(0.,0.,4.5));
#3779=CARTESIAN_POINT('',(-3.5,0.,4.5));
#3780=CARTESIAN_POINT('',(-3.5,0.,4.5));
#3781=CARTESIAN_POINT('Origin',(0.,0.,4.5));
#3782=CARTESIAN_POINT('Origin',(0.,0.,4.5));
#3783=CARTESIAN_POINT('',(-2.35,6.,4.5));
#3784=CARTESIAN_POINT('Origin',(0.,6.,4.5));
#3785=CARTESIAN_POINT('',(-2.35,0.,4.5));
#3786=CARTESIAN_POINT('',(-2.35,0.,4.5));
#3787=CARTESIAN_POINT('Origin',(0.,0.,4.5));
#3788=CARTESIAN_POINT('Origin',(0.,0.,4.5));
#3789=CARTESIAN_POINT('',(-3.5,6.,4.5));
#3790=CARTESIAN_POINT('Origin',(0.,6.,4.5));
#3791=CARTESIAN_POINT('',(-3.5,0.,4.5));
#3792=CARTESIAN_POINT('Origin',(0.,6.,4.5));
#3793=CARTESIAN_POINT('Origin',(0.,0.,4.5));
#5500=UNCERTAINTY_MEASURE_WITH_UNIT(LENGTH_MEASURE(0.001),#5536,
'DISTANCE_ACCURACY_VALUE',
'Maximum model space distance between geometric entities at asserted c
onnectivities');
#5516=UNCERTAINTY_MEASURE_WITH_UNIT(LENGTH_MEASURE(0.001),#5536,
'DISTANCE_ACCURACY_VALUE',
'Maximum model space distance between geometric entities at asserted c
onnectivities');
#5519=(
GEOMETRIC_REPRESENTATION_CONTEXT(3)
GLOBAL_UNCERTAINTY_ASSIGNED_CONTEXT((#5500))
GLOBAL_UNIT_ASSIGNED_CONTEXT((#5536,#5538,#5539))
REPRESENTATION_CONTEXT('','3D')
);
#5535=(
GEOMETRIC_REPRESENTATION_CONTEXT(3)
GLOBAL_UNCERTAINTY_ASSIGNED_CONTEXT((#5516))
GLOBAL_UNIT_ASSIGNED_CONTEXT((#5536,#5538,#5539))
REPRESENTATION_CONTEXT('','3D')
);
#5536=(
LENGTH_UNIT()
NAMED_UNIT(*)
SI_UNIT(.CENTI.,.METRE.)
);
#5538=(
NAMED_UNIT(*)
PLANE_ANGLE_UNIT()
SI_UNIT($,.RADIAN.)
);
#5539=(
NAMED_UNIT(*)
SI_UNIT($,.STERADIAN.)
SOLID_ANGLE_UNIT()
);
#5542=SHAPE_DEFINITION_REPRESENTATION(#5560,#5603);
#5560=PRODUCT_DEFINITION_SHAPE('',$,#5622);
#5603=SHAPE_REPRESENTATION('',(#2504),#5519);
#5619=PRODUCT_DEFINITION_CONTEXT('part definition',#5675,'design');
#5622=PRODUCT_DEFINITION('Flanged housing','Flanged housing',#5640,#5619);
#5640=PRODUCT_DEFINITION_FORMATION('',$,#5679);
#5675=APPLICATION_CONTEXT(
'Core Data for Automotive Mechanical Design Process');
#5676=PRODUCT_CONTEXT('part definition',#5675,'mechanical');
#5679=PRODUCT('Flanged housing','Flanged housing','Flanged housing',(#5676));
#5737=COLOUR_RGB('Dark Blue',0.08,0.2,0.34);
#5738=FILL_AREA_STYLE_COLOUR('',#5737);
#5739=FILL_AREA_STYLE('',(#5738));
#5740=SURFACE_STYLE_FILL_AREA(#5739);
#5741=SURFACE_SIDE_STYLE('',(#5740));
#5742=SURFACE_STYLE_USAGE(.BOTH.,#5741);
#5743=PRESENTATION_STYLE_ASSIGNMENT((#5742));
ENDSEC;
END-ISO-10303-21;
